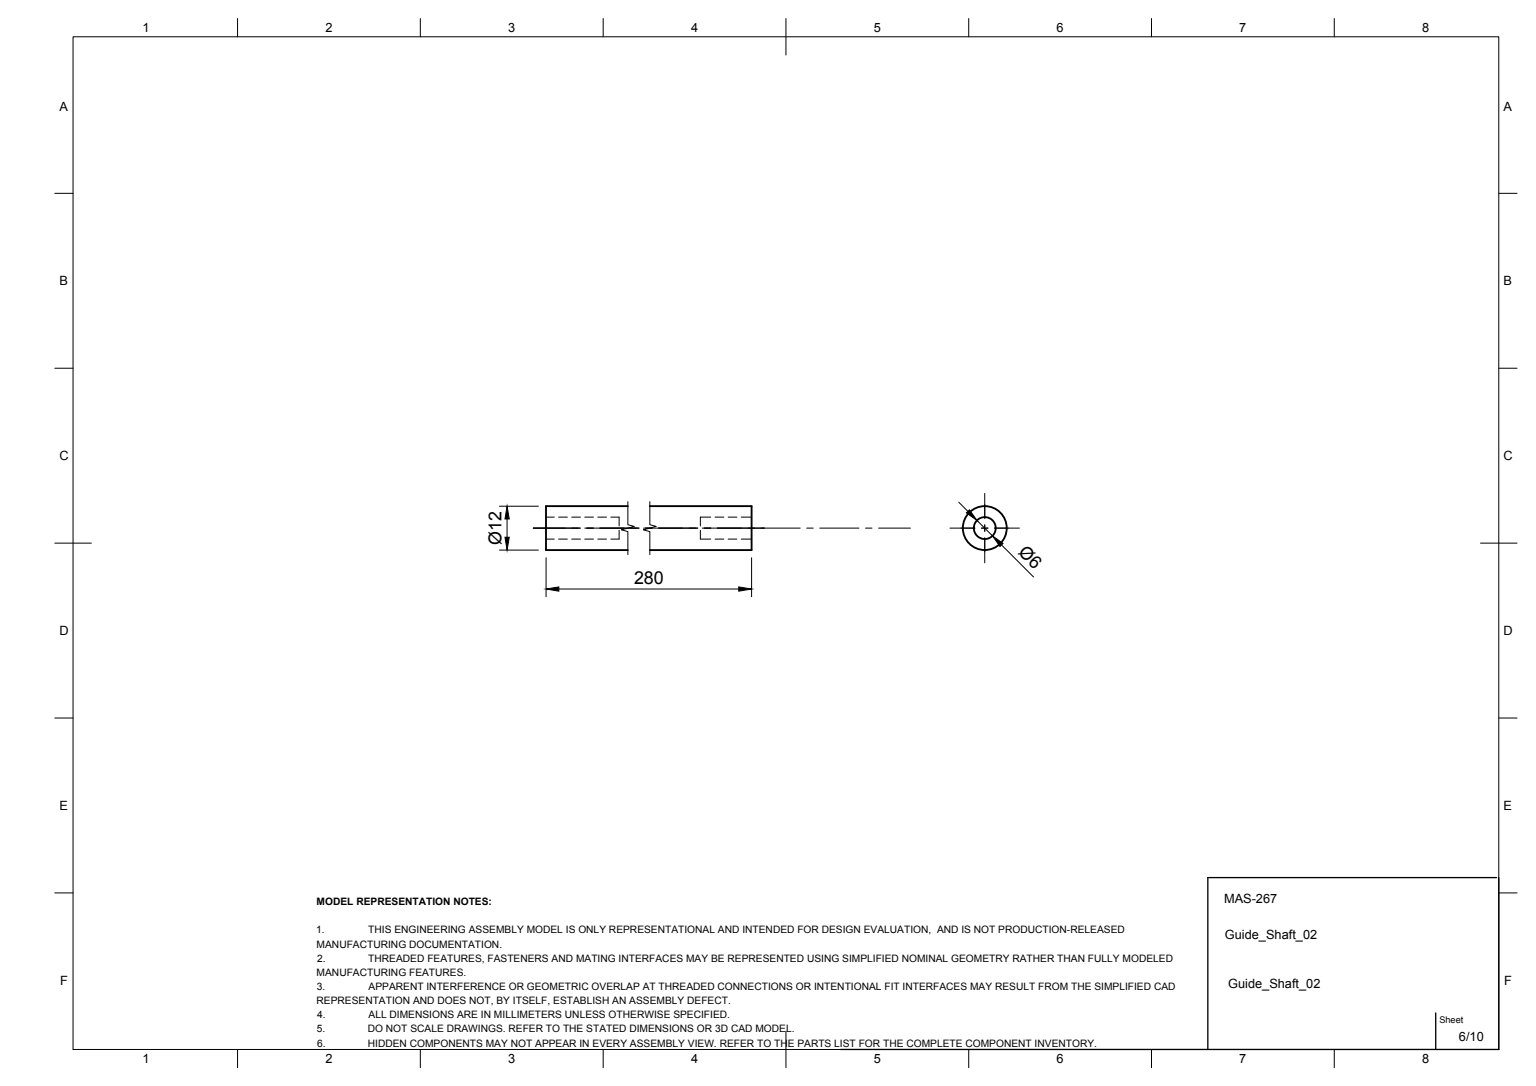
ISO-10303-21;
HEADER;
/* Generated by software containing ST-Developer
 * from STEP Tools, Inc. (www.steptools.com) 
 */

FILE_DESCRIPTION(
/* description */ (''),
/* implementation_level */ '2;1');

FILE_NAME(
/* name */ 'Guide_Shaft_02.step',
/* time_stamp */ '2026-10-12T15:29:24-07:00',
/* author */ (''),
/* organization */ (''),
/* preprocessor_version */ 'ST-DEVELOPER v20.2',
/* originating_system */ 'Autodesk Translation Framework v15.15.0.0',
/* authorisation */ '');

FILE_SCHEMA (('AUTOMOTIVE_DESIGN { 1 0 10303 214 3 1 1 }'));
ENDSEC;

DATA;
#10=MECHANICAL_DESIGN_GEOMETRIC_PRESENTATION_REPRESENTATION('',(#195),#9496);
#149=SHAPE_REPRESENTATION_RELATIONSHIP('SRR','None',#9543,#158);
#158=ADVANCED_BREP_SHAPE_REPRESENTATION('',(#252),#9491);
#195=STYLED_ITEM('',(#9594),#252);
#252=MANIFOLD_SOLID_BREP('Body1',#4997);
#414=FACE_BOUND('',#1242,.T.);
#415=FACE_BOUND('',#1245,.T.);
#560=PLANE('',#5546);
#561=PLANE('',#5550);
#562=PLANE('',#5551);
#563=PLANE('',#5555);
#824=FACE_OUTER_BOUND('',#1237,.T.);
#825=FACE_OUTER_BOUND('',#1238,.T.);
#826=FACE_OUTER_BOUND('',#1239,.T.);
#827=FACE_OUTER_BOUND('',#1240,.T.);
#828=FACE_OUTER_BOUND('',#1241,.T.);
#829=FACE_OUTER_BOUND('',#1243,.T.);
#830=FACE_OUTER_BOUND('',#1244,.T.);
#1237=EDGE_LOOP('',(#4029,#4030,#4031,#4032));
#1238=EDGE_LOOP('',(#4033));
#1239=EDGE_LOOP('',(#4034,#4035,#4036,#4037));
#1240=EDGE_LOOP('',(#4038));
#1241=EDGE_LOOP('',(#4039));
#1242=EDGE_LOOP('',(#4040));
#1243=EDGE_LOOP('',(#4041,#4042,#4043,#4044));
#1244=EDGE_LOOP('',(#4045));
#1245=EDGE_LOOP('',(#4046));
#1562=LINE('',#8600,#1799);
#1563=LINE('',#8607,#1800);
#1564=LINE('',#8615,#1801);
#1799=VECTOR('',#6799,3.);
#1800=VECTOR('',#6808,3.);
#1801=VECTOR('',#6819,6.00000000000001);
#2132=CIRCLE('',#5544,3.);
#2133=CIRCLE('',#5545,3.);
#2134=CIRCLE('',#5548,3.);
#2135=CIRCLE('',#5549,3.);
#2136=CIRCLE('',#5552,6.00000000000001);
#2137=CIRCLE('',#5554,6.00000000000001);
#2517=VERTEX_POINT('',#8597);
#2518=VERTEX_POINT('',#8599);
#2519=VERTEX_POINT('',#8604);
#2520=VERTEX_POINT('',#8606);
#2521=VERTEX_POINT('',#8611);
#2522=VERTEX_POINT('',#8614);
#3067=EDGE_CURVE('',#2517,#2517,#2132,.T.);
#3068=EDGE_CURVE('',#2517,#2518,#1562,.T.);
#3069=EDGE_CURVE('',#2518,#2518,#2133,.T.);
#3070=EDGE_CURVE('',#2519,#2519,#2134,.T.);
#3071=EDGE_CURVE('',#2519,#2520,#1563,.T.);
#3072=EDGE_CURVE('',#2520,#2520,#2135,.T.);
#3073=EDGE_CURVE('',#2521,#2521,#2136,.T.);
#3074=EDGE_CURVE('',#2521,#2522,#1564,.T.);
#3075=EDGE_CURVE('',#2522,#2522,#2137,.T.);
#4029=ORIENTED_EDGE('',*,*,#3067,.F.);
#4030=ORIENTED_EDGE('',*,*,#3068,.T.);
#4031=ORIENTED_EDGE('',*,*,#3069,.T.);
#4032=ORIENTED_EDGE('',*,*,#3068,.F.);
#4033=ORIENTED_EDGE('',*,*,#3069,.F.);
#4034=ORIENTED_EDGE('',*,*,#3070,.F.);
#4035=ORIENTED_EDGE('',*,*,#3071,.T.);
#4036=ORIENTED_EDGE('',*,*,#3072,.T.);
#4037=ORIENTED_EDGE('',*,*,#3071,.F.);
#4038=ORIENTED_EDGE('',*,*,#3072,.F.);
#4039=ORIENTED_EDGE('',*,*,#3073,.F.);
#4040=ORIENTED_EDGE('',*,*,#3067,.T.);
#4041=ORIENTED_EDGE('',*,*,#3073,.T.);
#4042=ORIENTED_EDGE('',*,*,#3074,.T.);
#4043=ORIENTED_EDGE('',*,*,#3075,.T.);
#4044=ORIENTED_EDGE('',*,*,#3074,.F.);
#4045=ORIENTED_EDGE('',*,*,#3075,.F.);
#4046=ORIENTED_EDGE('',*,*,#3070,.T.);
#4603=CYLINDRICAL_SURFACE('',#5543,3.);
#4604=CYLINDRICAL_SURFACE('',#5547,3.);
#4605=CYLINDRICAL_SURFACE('',#5553,6.00000000000001);
#4835=ADVANCED_FACE('',(#824),#4603,.F.);
#4836=ADVANCED_FACE('',(#825),#560,.T.);
#4837=ADVANCED_FACE('',(#826),#4604,.F.);
#4838=ADVANCED_FACE('',(#827),#561,.T.);
#4839=ADVANCED_FACE('',(#828,#414),#562,.T.);
#4840=ADVANCED_FACE('',(#829),#4605,.T.);
#4841=ADVANCED_FACE('',(#830,#415),#563,.F.);
#4997=CLOSED_SHELL('',(#4835,#4836,#4837,#4838,#4839,#4840,#4841));
#5542=AXIS2_PLACEMENT_3D('',#8595,#6793,#6794);
#5543=AXIS2_PLACEMENT_3D('',#8596,#6795,#6796);
#5544=AXIS2_PLACEMENT_3D('',#8598,#6797,#6798);
#5545=AXIS2_PLACEMENT_3D('',#8601,#6800,#6801);
#5546=AXIS2_PLACEMENT_3D('',#8602,#6802,#6803);
#5547=AXIS2_PLACEMENT_3D('',#8603,#6804,#6805);
#5548=AXIS2_PLACEMENT_3D('',#8605,#6806,#6807);
#5549=AXIS2_PLACEMENT_3D('',#8608,#6809,#6810);
#5550=AXIS2_PLACEMENT_3D('',#8609,#6811,#6812);
#5551=AXIS2_PLACEMENT_3D('',#8610,#6813,#6814);
#5552=AXIS2_PLACEMENT_3D('',#8612,#6815,#6816);
#5553=AXIS2_PLACEMENT_3D('',#8613,#6817,#6818);
#5554=AXIS2_PLACEMENT_3D('',#8616,#6820,#6821);
#5555=AXIS2_PLACEMENT_3D('',#8617,#6822,#6823);
#6793=DIRECTION('axis',(0.,0.,1.));
#6794=DIRECTION('refdir',(1.,0.,0.));
#6795=DIRECTION('center_axis',(1.,0.,0.));
#6796=DIRECTION('ref_axis',(0.,-1.,0.));
#6797=DIRECTION('center_axis',(1.,0.,0.));
#6798=DIRECTION('ref_axis',(0.,-1.,0.));
#6799=DIRECTION('',(1.,0.,0.));
#6800=DIRECTION('center_axis',(1.,0.,0.));
#6801=DIRECTION('ref_axis',(0.,-1.,0.));
#6802=DIRECTION('center_axis',(-1.,0.,0.));
#6803=DIRECTION('ref_axis',(0.,-1.,0.));
#6804=DIRECTION('center_axis',(-1.,0.,0.));
#6805=DIRECTION('ref_axis',(0.,1.,0.));
#6806=DIRECTION('center_axis',(-1.,0.,0.));
#6807=DIRECTION('ref_axis',(0.,1.,0.));
#6808=DIRECTION('',(-1.,0.,0.));
#6809=DIRECTION('center_axis',(-1.,0.,0.));
#6810=DIRECTION('ref_axis',(0.,1.,0.));
#6811=DIRECTION('center_axis',(1.,0.,0.));
#6812=DIRECTION('ref_axis',(0.,1.,0.));
#6813=DIRECTION('center_axis',(-1.,0.,0.));
#6814=DIRECTION('ref_axis',(0.,-1.,0.));
#6815=DIRECTION('center_axis',(1.,0.,0.));
#6816=DIRECTION('ref_axis',(0.,-1.,0.));
#6817=DIRECTION('center_axis',(-1.,0.,0.));
#6818=DIRECTION('ref_axis',(0.,-1.,0.));
#6819=DIRECTION('',(1.,0.,0.));
#6820=DIRECTION('center_axis',(-1.,0.,0.));
#6821=DIRECTION('ref_axis',(0.,-1.,0.));
#6822=DIRECTION('center_axis',(-1.,0.,0.));
#6823=DIRECTION('ref_axis',(0.,-1.,0.));
#8595=CARTESIAN_POINT('',(0.,0.,0.));
#8596=CARTESIAN_POINT('Origin',(-150.,37.8343839603864,-7.99999999999999));
#8597=CARTESIAN_POINT('',(-140.,40.8343839603864,-7.99999999999999));
#8598=CARTESIAN_POINT('Origin',(-140.,37.8343839603864,-7.99999999999999));
#8599=CARTESIAN_POINT('',(-126.,40.8343839603864,-7.99999999999999));
#8600=CARTESIAN_POINT('',(-150.,40.8343839603864,-7.99999999999999));
#8601=CARTESIAN_POINT('Origin',(-126.,37.8343839603864,-7.99999999999999));
#8602=CARTESIAN_POINT('Origin',(-126.,37.8343839603864,-7.99999999999999));
#8603=CARTESIAN_POINT('Origin',(150.,37.8343839603864,-8.00000000000001));
#8604=CARTESIAN_POINT('',(140.,34.8343839603864,-8.00000000000001));
#8605=CARTESIAN_POINT('Origin',(140.,37.8343839603864,-8.00000000000001));
#8606=CARTESIAN_POINT('',(120.,34.8343839603864,-8.00000000000001));
#8607=CARTESIAN_POINT('',(150.,34.8343839603864,-8.00000000000001));
#8608=CARTESIAN_POINT('Origin',(120.,37.8343839603864,-8.00000000000001));
#8609=CARTESIAN_POINT('Origin',(120.,37.8343839603864,-8.00000000000001));
#8610=CARTESIAN_POINT('Origin',(-140.,37.8343839603864,-7.99999999999999));
#8611=CARTESIAN_POINT('',(-140.,43.8343839603864,-7.99999999999999));
#8612=CARTESIAN_POINT('Origin',(-140.,37.8343839603864,-7.99999999999999));
#8613=CARTESIAN_POINT('Origin',(0.,37.8343839603864,-7.99999999999999));
#8614=CARTESIAN_POINT('',(140.,43.8343839603864,-7.99999999999999));
#8615=CARTESIAN_POINT('',(0.,43.8343839603864,-7.99999999999999));
#8616=CARTESIAN_POINT('Origin',(140.,37.8343839603864,-7.99999999999999));
#8617=CARTESIAN_POINT('Origin',(140.,37.8343839603864,-7.99999999999999));
#9480=UNCERTAINTY_MEASURE_WITH_UNIT(LENGTH_MEASURE(0.01),#9497,
'DISTANCE_ACCURACY_VALUE',
'Maximum model space distance between geometric entities at asserted c
onnectivities');
#9485=UNCERTAINTY_MEASURE_WITH_UNIT(LENGTH_MEASURE(0.01),#9497,
'DISTANCE_ACCURACY_VALUE',
'Maximum model space distance between geometric entities at asserted c
onnectivities');
#9491=(
GEOMETRIC_REPRESENTATION_CONTEXT(3)
GLOBAL_UNCERTAINTY_ASSIGNED_CONTEXT((#9480))
GLOBAL_UNIT_ASSIGNED_CONTEXT((#9497,#9499,#9500))
REPRESENTATION_CONTEXT('','3D')
);
#9496=(
GEOMETRIC_REPRESENTATION_CONTEXT(3)
GLOBAL_UNCERTAINTY_ASSIGNED_CONTEXT((#9485))
GLOBAL_UNIT_ASSIGNED_CONTEXT((#9497,#9499,#9500))
REPRESENTATION_CONTEXT('','3D')
);
#9497=(
LENGTH_UNIT()
NAMED_UNIT(*)
SI_UNIT(.MILLI.,.METRE.)
);
#9499=(
NAMED_UNIT(*)
PLANE_ANGLE_UNIT()
SI_UNIT($,.RADIAN.)
);
#9500=(
NAMED_UNIT(*)
SI_UNIT($,.STERADIAN.)
SOLID_ANGLE_UNIT()
);
#9506=SHAPE_DEFINITION_REPRESENTATION(#9516,#9543);
#9516=PRODUCT_DEFINITION_SHAPE('',$,#9554);
#9543=SHAPE_REPRESENTATION('',(#5542),#9491);
#9548=PRODUCT_DEFINITION_CONTEXT('part definition',#9580,'design');
#9554=PRODUCT_DEFINITION('Guide_Shaft_02','Guide_Shaft_02',#9564,#9548);
#9564=PRODUCT_DEFINITION_FORMATION('',$,#9587);
#9580=APPLICATION_CONTEXT(
'Core Data for Automotive Mechanical Design Process');
#9581=PRODUCT_CONTEXT('part definition',#9580,'mechanical');
#9587=PRODUCT('Guide_Shaft_02','Guide_Shaft_02',$,(#9581));
#9594=PRESENTATION_STYLE_ASSIGNMENT((#9597));
#9597=SURFACE_STYLE_USAGE(.BOTH.,#9600);
#9600=SURFACE_SIDE_STYLE('',(#9603));
#9603=SURFACE_STYLE_FILL_AREA(#9606);
#9606=FILL_AREA_STYLE('Opaque(160,160,160)',(#9609));
#9609=FILL_AREA_STYLE_COLOUR('Opaque(160,160,160)',#9612);
#9612=COLOUR_RGB('Opaque(160,160,160)', 0.40784314, 0.44705882, 0.49803922);
ENDSEC;
END-ISO-10303-21;
